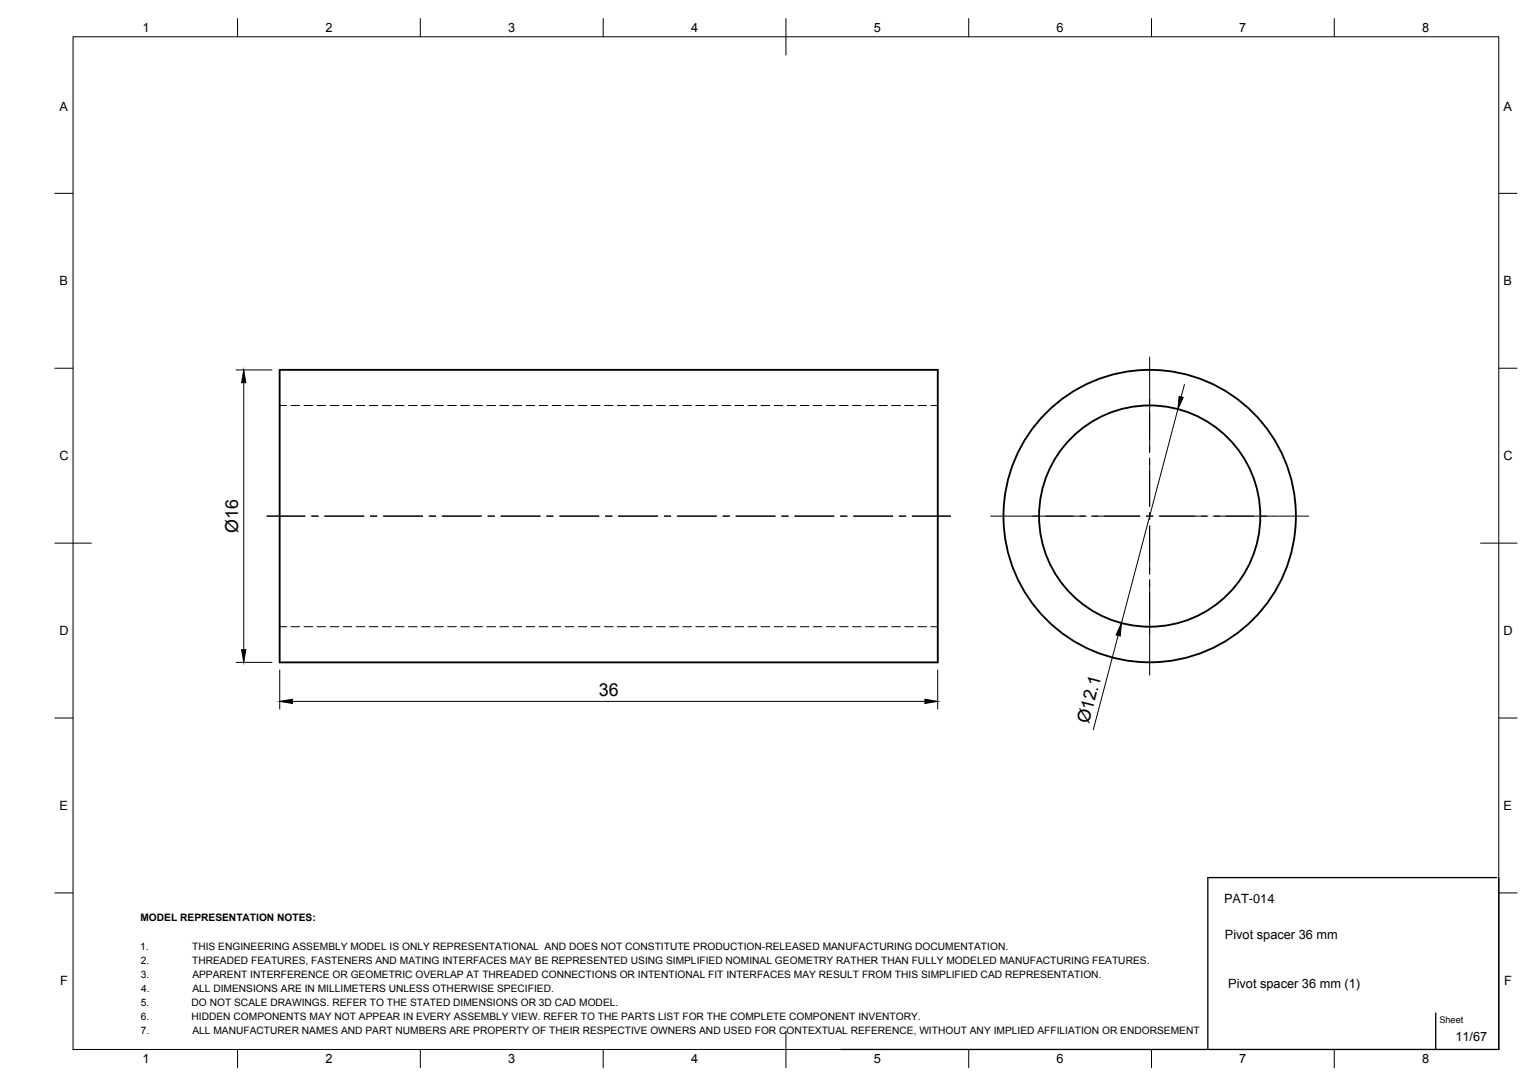
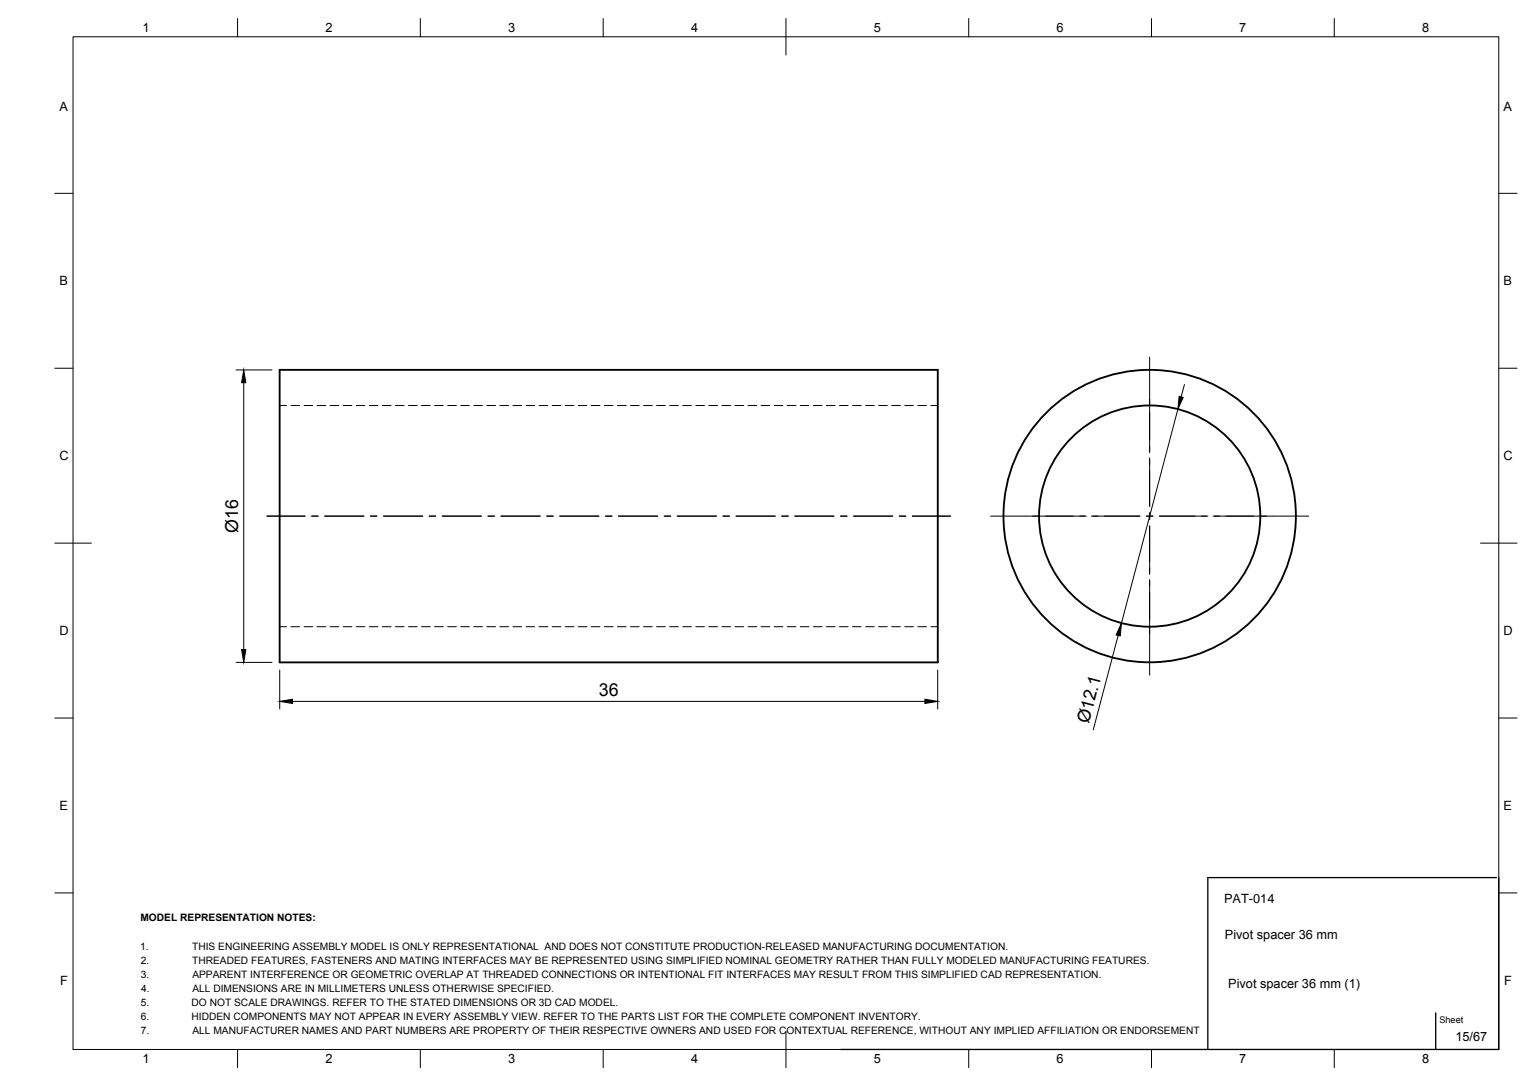
ISO-10303-21;
HEADER;
/* Generated by software containing ST-Developer
 * from STEP Tools, Inc. (www.steptools.com) 
 */

FILE_DESCRIPTION(
/* description */ ('Bin tilter linkage'),
/* implementation_level */ '2;1');

FILE_NAME(
/* name */ 'Pivot spacer 36 mm.step',
/* time_stamp */ '2026-10-28T03:26:24-07:00',
/* author */ (''),
/* organization */ (''),
/* preprocessor_version */ 'ST-DEVELOPER v20.2',
/* originating_system */ 'Autodesk Translation Framework v15.17.0.0',
/* authorisation */ '');

FILE_SCHEMA (('AUTOMOTIVE_DESIGN { 1 0 10303 214 3 1 1 }'));
ENDSEC;

DATA;
#10=MECHANICAL_DESIGN_GEOMETRIC_PRESENTATION_REPRESENTATION('',(#868),#23728);
#656=SHAPE_REPRESENTATION_RELATIONSHIP('SRR','None',#24120,#762);
#762=ADVANCED_BREP_SHAPE_REPRESENTATION('',(#982),#23620);
#868=STYLED_ITEM('',(#24758),#982);
#982=MANIFOLD_SOLID_BREP('Body1',#12398);
#1152=FACE_BOUND('',#2813,.T.);
#1153=FACE_BOUND('',#2815,.T.);
#1535=PLANE('',#13839);
#1536=PLANE('',#13840);
#1968=FACE_OUTER_BOUND('',#2810,.T.);
#1969=FACE_OUTER_BOUND('',#2811,.T.);
#1970=FACE_OUTER_BOUND('',#2812,.T.);
#1971=FACE_OUTER_BOUND('',#2814,.T.);
#2810=EDGE_LOOP('',(#8751,#8752,#8753,#8754));
#2811=EDGE_LOOP('',(#8755,#8756,#8757,#8758));
#2812=EDGE_LOOP('',(#8759));
#2813=EDGE_LOOP('',(#8760));
#2814=EDGE_LOOP('',(#8761));
#2815=EDGE_LOOP('',(#8762));
#3968=LINE('',#20151,#4643);
#3969=LINE('',#20157,#4644);
#4643=VECTOR('',#15911,0.605);
#4644=VECTOR('',#15918,0.8);
#5269=CIRCLE('',#13834,0.605);
#5270=CIRCLE('',#13835,0.605);
#5271=CIRCLE('',#13837,0.8);
#5272=CIRCLE('',#13838,0.8);
#6083=VERTEX_POINT('',#20148);
#6084=VERTEX_POINT('',#20150);
#6085=VERTEX_POINT('',#20154);
#6086=VERTEX_POINT('',#20156);
#7115=EDGE_CURVE('',#6083,#6083,#5269,.T.);
#7116=EDGE_CURVE('',#6083,#6084,#3968,.T.);
#7117=EDGE_CURVE('',#6084,#6084,#5270,.T.);
#7118=EDGE_CURVE('',#6085,#6085,#5271,.T.);
#7119=EDGE_CURVE('',#6085,#6086,#3969,.T.);
#7120=EDGE_CURVE('',#6086,#6086,#5272,.T.);
#8751=ORIENTED_EDGE('',*,*,#7115,.F.);
#8752=ORIENTED_EDGE('',*,*,#7116,.T.);
#8753=ORIENTED_EDGE('',*,*,#7117,.T.);
#8754=ORIENTED_EDGE('',*,*,#7116,.F.);
#8755=ORIENTED_EDGE('',*,*,#7118,.F.);
#8756=ORIENTED_EDGE('',*,*,#7119,.T.);
#8757=ORIENTED_EDGE('',*,*,#7120,.T.);
#8758=ORIENTED_EDGE('',*,*,#7119,.F.);
#8759=ORIENTED_EDGE('',*,*,#7118,.T.);
#8760=ORIENTED_EDGE('',*,*,#7115,.T.);
#8761=ORIENTED_EDGE('',*,*,#7120,.F.);
#8762=ORIENTED_EDGE('',*,*,#7117,.F.);
#11302=CYLINDRICAL_SURFACE('',#13833,0.605);
#11303=CYLINDRICAL_SURFACE('',#13836,0.8);
#11693=ADVANCED_FACE('',(#1968),#11302,.F.);
#11694=ADVANCED_FACE('',(#1969),#11303,.T.);
#11695=ADVANCED_FACE('',(#1970,#1152),#1535,.T.);
#11696=ADVANCED_FACE('',(#1971,#1153),#1536,.F.);
#12398=CLOSED_SHELL('',(#11693,#11694,#11695,#11696));
#13832=AXIS2_PLACEMENT_3D('',#20146,#15905,#15906);
#13833=AXIS2_PLACEMENT_3D('',#20147,#15907,#15908);
#13834=AXIS2_PLACEMENT_3D('',#20149,#15909,#15910);
#13835=AXIS2_PLACEMENT_3D('',#20152,#15912,#15913);
#13836=AXIS2_PLACEMENT_3D('',#20153,#15914,#15915);
#13837=AXIS2_PLACEMENT_3D('',#20155,#15916,#15917);
#13838=AXIS2_PLACEMENT_3D('',#20158,#15919,#15920);
#13839=AXIS2_PLACEMENT_3D('',#20159,#15921,#15922);
#13840=AXIS2_PLACEMENT_3D('',#20160,#15923,#15924);
#15905=DIRECTION('axis',(0.,0.,1.));
#15906=DIRECTION('refdir',(1.,0.,0.));
#15907=DIRECTION('center_axis',(0.,1.,0.));
#15908=DIRECTION('ref_axis',(1.,0.,0.));
#15909=DIRECTION('center_axis',(0.,-1.,0.));
#15910=DIRECTION('ref_axis',(1.,0.,0.));
#15911=DIRECTION('',(0.,-1.,0.));
#15912=DIRECTION('center_axis',(0.,-1.,0.));
#15913=DIRECTION('ref_axis',(1.,0.,0.));
#15914=DIRECTION('center_axis',(0.,1.,0.));
#15915=DIRECTION('ref_axis',(1.,0.,0.));
#15916=DIRECTION('center_axis',(0.,1.,0.));
#15917=DIRECTION('ref_axis',(1.,0.,0.));
#15918=DIRECTION('',(0.,-1.,0.));
#15919=DIRECTION('center_axis',(0.,1.,0.));
#15920=DIRECTION('ref_axis',(1.,0.,0.));
#15921=DIRECTION('center_axis',(0.,1.,0.));
#15922=DIRECTION('ref_axis',(1.,0.,0.));
#15923=DIRECTION('center_axis',(0.,1.,0.));
#15924=DIRECTION('ref_axis',(1.,0.,0.));
#20146=CARTESIAN_POINT('',(0.,0.,0.));
#20147=CARTESIAN_POINT('Origin',(0.,0.5,15.));
#20148=CARTESIAN_POINT('',(-0.605,4.1,15.));
#20149=CARTESIAN_POINT('Origin',(0.,4.1,15.));
#20150=CARTESIAN_POINT('',(-0.605,0.5,15.));
#20151=CARTESIAN_POINT('',(-0.605,0.5,15.));
#20152=CARTESIAN_POINT('Origin',(0.,0.5,15.));
#20153=CARTESIAN_POINT('Origin',(0.,0.5,15.));
#20154=CARTESIAN_POINT('',(-0.8,4.1,15.));
#20155=CARTESIAN_POINT('Origin',(0.,4.1,15.));
#20156=CARTESIAN_POINT('',(-0.8,0.5,15.));
#20157=CARTESIAN_POINT('',(-0.8,0.5,15.));
#20158=CARTESIAN_POINT('Origin',(0.,0.5,15.));
#20159=CARTESIAN_POINT('Origin',(0.,4.1,15.));
#20160=CARTESIAN_POINT('Origin',(0.,0.5,15.));
#23503=UNCERTAINTY_MEASURE_WITH_UNIT(LENGTH_MEASURE(0.001),#23729,
'DISTANCE_ACCURACY_VALUE',
'Maximum model space distance between geometric entities at asserted c
onnectivities');
#23611=UNCERTAINTY_MEASURE_WITH_UNIT(LENGTH_MEASURE(0.001),#23729,
'DISTANCE_ACCURACY_VALUE',
'Maximum model space distance between geometric entities at asserted c
onnectivities');
#23620=(
GEOMETRIC_REPRESENTATION_CONTEXT(3)
GLOBAL_UNCERTAINTY_ASSIGNED_CONTEXT((#23503))
GLOBAL_UNIT_ASSIGNED_CONTEXT((#23729,#23731,#23732))
REPRESENTATION_CONTEXT('','3D')
);
#23728=(
GEOMETRIC_REPRESENTATION_CONTEXT(3)
GLOBAL_UNCERTAINTY_ASSIGNED_CONTEXT((#23611))
GLOBAL_UNIT_ASSIGNED_CONTEXT((#23729,#23731,#23732))
REPRESENTATION_CONTEXT('','3D')
);
#23729=(
LENGTH_UNIT()
NAMED_UNIT(*)
SI_UNIT(.CENTI.,.METRE.)
);
#23731=(
NAMED_UNIT(*)
PLANE_ANGLE_UNIT()
SI_UNIT($,.RADIAN.)
);
#23732=(
NAMED_UNIT(*)
SI_UNIT($,.STERADIAN.)
SOLID_ANGLE_UNIT()
);
#23741=SHAPE_DEFINITION_REPRESENTATION(#23857,#24120);
#23857=PRODUCT_DEFINITION_SHAPE('',$,#24237);
#24120=SHAPE_REPRESENTATION('',(#13832),#23620);
#24228=PRODUCT_DEFINITION_CONTEXT('part definition',#24578,'design');
#24237=PRODUCT_DEFINITION('Pivot spacer 36 mm','Pivot spacer 36 mm',#24353,
#24228);
#24353=PRODUCT_DEFINITION_FORMATION('',$,#24588);
#24578=APPLICATION_CONTEXT(
'Core Data for Automotive Mechanical Design Process');
#24579=PRODUCT_CONTEXT('part definition',#24578,'mechanical');
#24588=PRODUCT('Pivot spacer 36 mm','Pivot spacer 36 mm',
'Pivot spacer 36 mm',(#24579));
#24752=COLOUR_RGB('Sky Blue',0.24,0.69,0.87);
#24753=FILL_AREA_STYLE_COLOUR('',#24752);
#24754=FILL_AREA_STYLE('',(#24753));
#24755=SURFACE_STYLE_FILL_AREA(#24754);
#24756=SURFACE_SIDE_STYLE('',(#24755));
#24757=SURFACE_STYLE_USAGE(.BOTH.,#24756);
#24758=PRESENTATION_STYLE_ASSIGNMENT((#24757));
ENDSEC;
END-ISO-10303-21;
